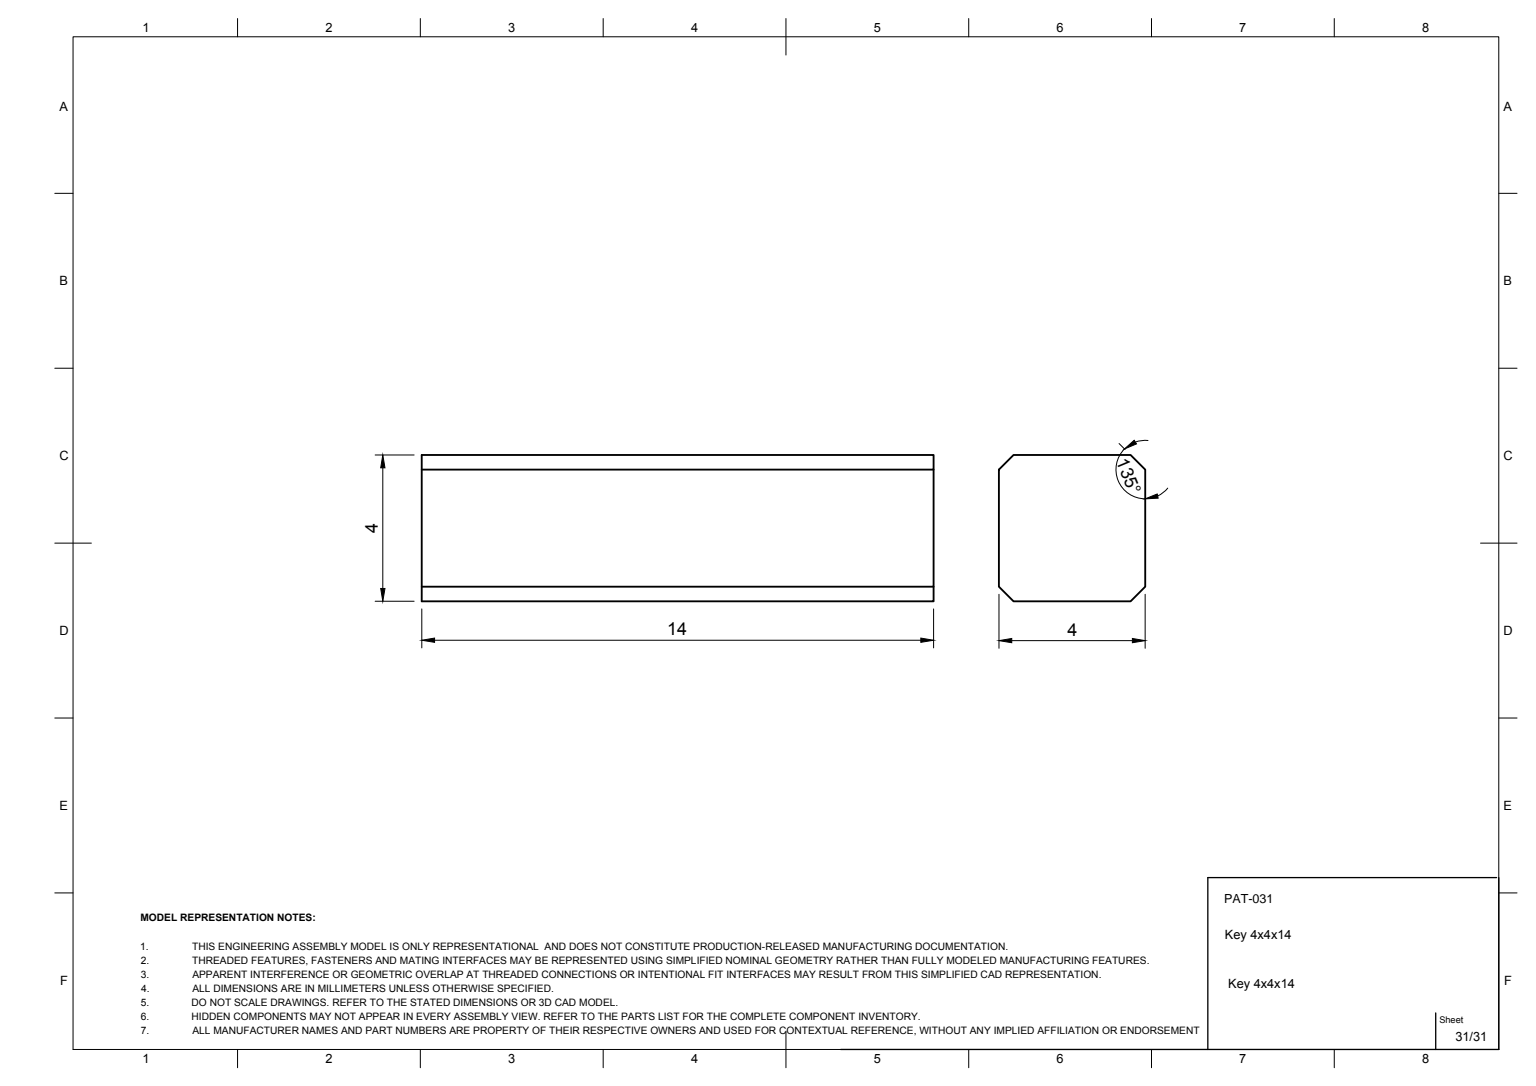
ISO-10303-21;
HEADER;
/* Generated by software containing ST-Developer
 * from STEP Tools, Inc. (www.steptools.com) 
 */

FILE_DESCRIPTION(
/* description */ ('Double-row support with tensioned shaft'),
/* implementation_level */ '2;1');

FILE_NAME(
/* name */ 'Key 4x4x14.step',
/* time_stamp */ '2026-10-27T10:50:35-07:00',
/* author */ (''),
/* organization */ (''),
/* preprocessor_version */ 'ST-DEVELOPER v20.2',
/* originating_system */ 'Autodesk Translation Framework v15.17.0.0',
/* authorisation */ '');

FILE_SCHEMA (('AUTOMOTIVE_DESIGN { 1 0 10303 214 3 1 1 }'));
ENDSEC;

DATA;
#10=MECHANICAL_DESIGN_GEOMETRIC_PRESENTATION_REPRESENTATION('',(#510),#11559);
#445=SHAPE_REPRESENTATION_RELATIONSHIP('SRR','None',#11755,#477);
#477=ADVANCED_BREP_SHAPE_REPRESENTATION('',(#540),#11557);
#510=STYLED_ITEM('',(#11967),#540);
#540=MANIFOLD_SOLID_BREP('Body1',#6358);
#898=PLANE('',#7334);
#899=PLANE('',#7335);
#900=PLANE('',#7336);
#901=PLANE('',#7337);
#902=PLANE('',#7338);
#903=PLANE('',#7339);
#904=PLANE('',#7340);
#905=PLANE('',#7341);
#906=PLANE('',#7342);
#907=PLANE('',#7343);
#1239=FACE_OUTER_BOUND('',#1719,.T.);
#1240=FACE_OUTER_BOUND('',#1720,.T.);
#1241=FACE_OUTER_BOUND('',#1721,.T.);
#1242=FACE_OUTER_BOUND('',#1722,.T.);
#1243=FACE_OUTER_BOUND('',#1723,.T.);
#1244=FACE_OUTER_BOUND('',#1724,.T.);
#1245=FACE_OUTER_BOUND('',#1725,.T.);
#1246=FACE_OUTER_BOUND('',#1726,.T.);
#1247=FACE_OUTER_BOUND('',#1727,.T.);
#1248=FACE_OUTER_BOUND('',#1728,.T.);
#1719=EDGE_LOOP('',(#5792,#5793,#5794,#5795,#5796,#5797,#5798,#5799));
#1720=EDGE_LOOP('',(#5800,#5801,#5802,#5803));
#1721=EDGE_LOOP('',(#5804,#5805,#5806,#5807));
#1722=EDGE_LOOP('',(#5808,#5809,#5810,#5811));
#1723=EDGE_LOOP('',(#5812,#5813,#5814,#5815));
#1724=EDGE_LOOP('',(#5816,#5817,#5818,#5819,#5820,#5821,#5822,#5823));
#1725=EDGE_LOOP('',(#5824,#5825,#5826,#5827));
#1726=EDGE_LOOP('',(#5828,#5829,#5830,#5831));
#1727=EDGE_LOOP('',(#5832,#5833,#5834,#5835));
#1728=EDGE_LOOP('',(#5836,#5837,#5838,#5839));
#2244=LINE('',#11375,#2791);
#2245=LINE('',#11377,#2792);
#2246=LINE('',#11379,#2793);
#2247=LINE('',#11381,#2794);
#2248=LINE('',#11383,#2795);
#2249=LINE('',#11385,#2796);
#2250=LINE('',#11387,#2797);
#2251=LINE('',#11388,#2798);
#2252=LINE('',#11391,#2799);
#2253=LINE('',#11393,#2800);
#2254=LINE('',#11394,#2801);
#2255=LINE('',#11397,#2802);
#2256=LINE('',#11398,#2803);
#2257=LINE('',#11401,#2804);
#2258=LINE('',#11402,#2805);
#2259=LINE('',#11405,#2806);
#2260=LINE('',#11406,#2807);
#2261=LINE('',#11409,#2808);
#2262=LINE('',#11411,#2809);
#2263=LINE('',#11413,#2810);
#2264=LINE('',#11414,#2811);
#2265=LINE('',#11416,#2812);
#2266=LINE('',#11418,#2813);
#2267=LINE('',#11420,#2814);
#2791=VECTOR('',#9117,1.);
#2792=VECTOR('',#9118,1.);
#2793=VECTOR('',#9119,1.);
#2794=VECTOR('',#9120,1.);
#2795=VECTOR('',#9121,1.);
#2796=VECTOR('',#9122,1.);
#2797=VECTOR('',#9123,1.);
#2798=VECTOR('',#9124,1.);
#2799=VECTOR('',#9127,1.);
#2800=VECTOR('',#9128,1.);
#2801=VECTOR('',#9129,1.);
#2802=VECTOR('',#9132,1.);
#2803=VECTOR('',#9133,1.);
#2804=VECTOR('',#9136,1.);
#2805=VECTOR('',#9137,1.);
#2806=VECTOR('',#9140,1.);
#2807=VECTOR('',#9141,1.);
#2808=VECTOR('',#9144,1.);
#2809=VECTOR('',#9145,1.);
#2810=VECTOR('',#9146,1.);
#2811=VECTOR('',#9147,1.);
#2812=VECTOR('',#9150,1.);
#2813=VECTOR('',#9153,1.);
#2814=VECTOR('',#9156,1.);
#3518=VERTEX_POINT('',#11373);
#3519=VERTEX_POINT('',#11374);
#3520=VERTEX_POINT('',#11376);
#3521=VERTEX_POINT('',#11378);
#3522=VERTEX_POINT('',#11380);
#3523=VERTEX_POINT('',#11382);
#3524=VERTEX_POINT('',#11384);
#3525=VERTEX_POINT('',#11386);
#3526=VERTEX_POINT('',#11390);
#3527=VERTEX_POINT('',#11392);
#3528=VERTEX_POINT('',#11396);
#3529=VERTEX_POINT('',#11400);
#3530=VERTEX_POINT('',#11404);
#3531=VERTEX_POINT('',#11408);
#3532=VERTEX_POINT('',#11410);
#3533=VERTEX_POINT('',#11412);
#4281=EDGE_CURVE('',#3518,#3519,#2244,.T.);
#4282=EDGE_CURVE('',#3520,#3518,#2245,.T.);
#4283=EDGE_CURVE('',#3521,#3520,#2246,.T.);
#4284=EDGE_CURVE('',#3522,#3521,#2247,.T.);
#4285=EDGE_CURVE('',#3523,#3522,#2248,.T.);
#4286=EDGE_CURVE('',#3524,#3523,#2249,.T.);
#4287=EDGE_CURVE('',#3525,#3524,#2250,.T.);
#4288=EDGE_CURVE('',#3519,#3525,#2251,.T.);
#4289=EDGE_CURVE('',#3522,#3526,#2252,.T.);
#4290=EDGE_CURVE('',#3526,#3527,#2253,.T.);
#4291=EDGE_CURVE('',#3527,#3523,#2254,.T.);
#4292=EDGE_CURVE('',#3528,#3521,#2255,.T.);
#4293=EDGE_CURVE('',#3528,#3526,#2256,.T.);
#4294=EDGE_CURVE('',#3520,#3529,#2257,.T.);
#4295=EDGE_CURVE('',#3529,#3528,#2258,.T.);
#4296=EDGE_CURVE('',#3530,#3518,#2259,.T.);
#4297=EDGE_CURVE('',#3530,#3529,#2260,.T.);
#4298=EDGE_CURVE('',#3531,#3530,#2261,.T.);
#4299=EDGE_CURVE('',#3532,#3531,#2262,.T.);
#4300=EDGE_CURVE('',#3533,#3532,#2263,.T.);
#4301=EDGE_CURVE('',#3527,#3533,#2264,.T.);
#4302=EDGE_CURVE('',#3519,#3531,#2265,.T.);
#4303=EDGE_CURVE('',#3532,#3525,#2266,.T.);
#4304=EDGE_CURVE('',#3524,#3533,#2267,.T.);
#5792=ORIENTED_EDGE('',*,*,#4281,.F.);
#5793=ORIENTED_EDGE('',*,*,#4282,.F.);
#5794=ORIENTED_EDGE('',*,*,#4283,.F.);
#5795=ORIENTED_EDGE('',*,*,#4284,.F.);
#5796=ORIENTED_EDGE('',*,*,#4285,.F.);
#5797=ORIENTED_EDGE('',*,*,#4286,.F.);
#5798=ORIENTED_EDGE('',*,*,#4287,.F.);
#5799=ORIENTED_EDGE('',*,*,#4288,.F.);
#5800=ORIENTED_EDGE('',*,*,#4285,.T.);
#5801=ORIENTED_EDGE('',*,*,#4289,.T.);
#5802=ORIENTED_EDGE('',*,*,#4290,.T.);
#5803=ORIENTED_EDGE('',*,*,#4291,.T.);
#5804=ORIENTED_EDGE('',*,*,#4284,.T.);
#5805=ORIENTED_EDGE('',*,*,#4292,.F.);
#5806=ORIENTED_EDGE('',*,*,#4293,.T.);
#5807=ORIENTED_EDGE('',*,*,#4289,.F.);
#5808=ORIENTED_EDGE('',*,*,#4283,.T.);
#5809=ORIENTED_EDGE('',*,*,#4294,.T.);
#5810=ORIENTED_EDGE('',*,*,#4295,.T.);
#5811=ORIENTED_EDGE('',*,*,#4292,.T.);
#5812=ORIENTED_EDGE('',*,*,#4282,.T.);
#5813=ORIENTED_EDGE('',*,*,#4296,.F.);
#5814=ORIENTED_EDGE('',*,*,#4297,.T.);
#5815=ORIENTED_EDGE('',*,*,#4294,.F.);
#5816=ORIENTED_EDGE('',*,*,#4290,.F.);
#5817=ORIENTED_EDGE('',*,*,#4293,.F.);
#5818=ORIENTED_EDGE('',*,*,#4295,.F.);
#5819=ORIENTED_EDGE('',*,*,#4297,.F.);
#5820=ORIENTED_EDGE('',*,*,#4298,.F.);
#5821=ORIENTED_EDGE('',*,*,#4299,.F.);
#5822=ORIENTED_EDGE('',*,*,#4300,.F.);
#5823=ORIENTED_EDGE('',*,*,#4301,.F.);
#5824=ORIENTED_EDGE('',*,*,#4281,.T.);
#5825=ORIENTED_EDGE('',*,*,#4302,.T.);
#5826=ORIENTED_EDGE('',*,*,#4298,.T.);
#5827=ORIENTED_EDGE('',*,*,#4296,.T.);
#5828=ORIENTED_EDGE('',*,*,#4288,.T.);
#5829=ORIENTED_EDGE('',*,*,#4303,.F.);
#5830=ORIENTED_EDGE('',*,*,#4299,.T.);
#5831=ORIENTED_EDGE('',*,*,#4302,.F.);
#5832=ORIENTED_EDGE('',*,*,#4287,.T.);
#5833=ORIENTED_EDGE('',*,*,#4304,.T.);
#5834=ORIENTED_EDGE('',*,*,#4300,.T.);
#5835=ORIENTED_EDGE('',*,*,#4303,.T.);
#5836=ORIENTED_EDGE('',*,*,#4286,.T.);
#5837=ORIENTED_EDGE('',*,*,#4291,.F.);
#5838=ORIENTED_EDGE('',*,*,#4301,.T.);
#5839=ORIENTED_EDGE('',*,*,#4304,.F.);
#6302=ADVANCED_FACE('',(#1239),#898,.T.);
#6303=ADVANCED_FACE('',(#1240),#899,.T.);
#6304=ADVANCED_FACE('',(#1241),#900,.T.);
#6305=ADVANCED_FACE('',(#1242),#901,.T.);
#6306=ADVANCED_FACE('',(#1243),#902,.T.);
#6307=ADVANCED_FACE('',(#1244),#903,.F.);
#6308=ADVANCED_FACE('',(#1245),#904,.T.);
#6309=ADVANCED_FACE('',(#1246),#905,.T.);
#6310=ADVANCED_FACE('',(#1247),#906,.T.);
#6311=ADVANCED_FACE('',(#1248),#907,.F.);
#6358=CLOSED_SHELL('',(#6302,#6303,#6304,#6305,#6306,#6307,#6308,#6309,
#6310,#6311));
#7333=AXIS2_PLACEMENT_3D('',#11371,#9113,#9114);
#7334=AXIS2_PLACEMENT_3D('',#11372,#9115,#9116);
#7335=AXIS2_PLACEMENT_3D('',#11389,#9125,#9126);
#7336=AXIS2_PLACEMENT_3D('',#11395,#9130,#9131);
#7337=AXIS2_PLACEMENT_3D('',#11399,#9134,#9135);
#7338=AXIS2_PLACEMENT_3D('',#11403,#9138,#9139);
#7339=AXIS2_PLACEMENT_3D('',#11407,#9142,#9143);
#7340=AXIS2_PLACEMENT_3D('',#11415,#9148,#9149);
#7341=AXIS2_PLACEMENT_3D('',#11417,#9151,#9152);
#7342=AXIS2_PLACEMENT_3D('',#11419,#9154,#9155);
#7343=AXIS2_PLACEMENT_3D('',#11421,#9157,#9158);
#9113=DIRECTION('axis',(0.,0.,1.));
#9114=DIRECTION('refdir',(1.,0.,0.));
#9115=DIRECTION('center_axis',(1.,0.,0.));
#9116=DIRECTION('ref_axis',(0.,0.,-1.));
#9117=DIRECTION('',(0.,0.707106781186547,-0.707106781186548));
#9118=DIRECTION('',(0.,1.,0.));
#9119=DIRECTION('',(0.,0.707106781186547,0.707106781186548));
#9120=DIRECTION('',(0.,0.,1.));
#9121=DIRECTION('',(0.,-0.707106781186548,0.707106781186548));
#9122=DIRECTION('',(0.,-1.,0.));
#9123=DIRECTION('',(0.,-0.707106781186548,-0.707106781186548));
#9124=DIRECTION('',(0.,0.,-1.));
#9125=DIRECTION('center_axis',(0.,-0.707106781186548,-0.707106781186548));
#9126=DIRECTION('ref_axis',(-1.,0.,0.));
#9127=DIRECTION('',(-1.,0.,0.));
#9128=DIRECTION('',(0.,0.707106781186548,-0.707106781186548));
#9129=DIRECTION('',(1.,0.,0.));
#9130=DIRECTION('center_axis',(0.,-1.,0.));
#9131=DIRECTION('ref_axis',(1.,0.,0.));
#9132=DIRECTION('',(1.,0.,0.));
#9133=DIRECTION('',(0.,0.,-1.));
#9134=DIRECTION('center_axis',(0.,-0.707106781186548,0.707106781186547));
#9135=DIRECTION('ref_axis',(1.,0.,0.));
#9136=DIRECTION('',(-1.,0.,0.));
#9137=DIRECTION('',(0.,-0.707106781186547,-0.707106781186548));
#9138=DIRECTION('center_axis',(0.,0.,1.));
#9139=DIRECTION('ref_axis',(1.,0.,0.));
#9140=DIRECTION('',(1.,0.,0.));
#9141=DIRECTION('',(0.,-1.,0.));
#9142=DIRECTION('center_axis',(1.,0.,0.));
#9143=DIRECTION('ref_axis',(0.,0.,-1.));
#9144=DIRECTION('',(0.,-0.707106781186547,0.707106781186548));
#9145=DIRECTION('',(0.,0.,1.));
#9146=DIRECTION('',(0.,0.707106781186548,0.707106781186548));
#9147=DIRECTION('',(0.,1.,0.));
#9148=DIRECTION('center_axis',(0.,0.707106781186548,0.707106781186547));
#9149=DIRECTION('ref_axis',(1.,0.,0.));
#9150=DIRECTION('',(-1.,0.,0.));
#9151=DIRECTION('center_axis',(0.,1.,0.));
#9152=DIRECTION('ref_axis',(-1.,0.,0.));
#9153=DIRECTION('',(1.,0.,0.));
#9154=DIRECTION('center_axis',(0.,0.707106781186548,-0.707106781186548));
#9155=DIRECTION('ref_axis',(-1.,0.,0.));
#9156=DIRECTION('',(-1.,0.,0.));
#9157=DIRECTION('center_axis',(0.,0.,1.));
#9158=DIRECTION('ref_axis',(1.,0.,0.));
#11371=CARTESIAN_POINT('',(0.,0.,0.));
#11372=CARTESIAN_POINT('Origin',(0.7,0.,0.25));
#11373=CARTESIAN_POINT('',(0.7,0.16,0.4));
#11374=CARTESIAN_POINT('',(0.7,0.2,0.36));
#11375=CARTESIAN_POINT('',(0.7,0.1675,0.3925));
#11376=CARTESIAN_POINT('',(0.7,-0.16,0.4));
#11377=CARTESIAN_POINT('',(0.7,0.,0.4));
#11378=CARTESIAN_POINT('',(0.7,-0.2,0.36));
#11379=CARTESIAN_POINT('',(0.7,-0.1675,0.3925));
#11380=CARTESIAN_POINT('',(0.7,-0.2,0.04));
#11381=CARTESIAN_POINT('',(0.7,-0.2,0.125));
#11382=CARTESIAN_POINT('',(0.7,-0.16,0.));
#11383=CARTESIAN_POINT('',(0.7,-0.1925,0.0325));
#11384=CARTESIAN_POINT('',(0.7,0.16,0.));
#11385=CARTESIAN_POINT('',(0.7,0.,0.));
#11386=CARTESIAN_POINT('',(0.7,0.2,0.04));
#11387=CARTESIAN_POINT('',(0.7,0.1925,0.0325));
#11388=CARTESIAN_POINT('',(0.7,0.2,0.125));
#11389=CARTESIAN_POINT('Origin',(-0.4,-0.18,0.02));
#11390=CARTESIAN_POINT('',(-0.7,-0.2,0.04));
#11391=CARTESIAN_POINT('',(-0.4,-0.2,0.04));
#11392=CARTESIAN_POINT('',(-0.7,-0.16,0.));
#11393=CARTESIAN_POINT('',(-0.7,-0.1925,0.0325));
#11394=CARTESIAN_POINT('',(-0.4,-0.16,0.));
#11395=CARTESIAN_POINT('Origin',(-0.8,-0.2,0.));
#11396=CARTESIAN_POINT('',(-0.7,-0.2,0.36));
#11397=CARTESIAN_POINT('',(-0.4,-0.2,0.36));
#11398=CARTESIAN_POINT('',(-0.7,-0.2,0.125));
#11399=CARTESIAN_POINT('Origin',(-0.4,-0.18,0.38));
#11400=CARTESIAN_POINT('',(-0.7,-0.16,0.4));
#11401=CARTESIAN_POINT('',(-0.4,-0.16,0.4));
#11402=CARTESIAN_POINT('',(-0.7,-0.1675,0.3925));
#11403=CARTESIAN_POINT('Origin',(0.,0.,0.4));
#11404=CARTESIAN_POINT('',(-0.7,0.16,0.4));
#11405=CARTESIAN_POINT('',(0.4,0.16,0.4));
#11406=CARTESIAN_POINT('',(-0.7,0.,0.4));
#11407=CARTESIAN_POINT('Origin',(-0.7,0.,0.25));
#11408=CARTESIAN_POINT('',(-0.7,0.2,0.36));
#11409=CARTESIAN_POINT('',(-0.7,0.1675,0.3925));
#11410=CARTESIAN_POINT('',(-0.7,0.2,0.04));
#11411=CARTESIAN_POINT('',(-0.7,0.2,0.125));
#11412=CARTESIAN_POINT('',(-0.7,0.16,0.));
#11413=CARTESIAN_POINT('',(-0.7,0.1925,0.0325));
#11414=CARTESIAN_POINT('',(-0.7,0.,0.));
#11415=CARTESIAN_POINT('Origin',(0.4,0.18,0.38));
#11416=CARTESIAN_POINT('',(0.4,0.2,0.36));
#11417=CARTESIAN_POINT('Origin',(0.8,0.2,0.));
#11418=CARTESIAN_POINT('',(0.4,0.2,0.04));
#11419=CARTESIAN_POINT('Origin',(0.4,0.18,0.02));
#11420=CARTESIAN_POINT('',(0.4,0.16,0.));
#11421=CARTESIAN_POINT('Origin',(0.,0.,0.));
#11520=UNCERTAINTY_MEASURE_WITH_UNIT(LENGTH_MEASURE(0.001),#11560,
'DISTANCE_ACCURACY_VALUE',
'Maximum model space distance between geometric entities at asserted c
onnectivities');
#11522=UNCERTAINTY_MEASURE_WITH_UNIT(LENGTH_MEASURE(0.001),#11560,
'DISTANCE_ACCURACY_VALUE',
'Maximum model space distance between geometric entities at asserted c
onnectivities');
#11557=(
GEOMETRIC_REPRESENTATION_CONTEXT(3)
GLOBAL_UNCERTAINTY_ASSIGNED_CONTEXT((#11520))
GLOBAL_UNIT_ASSIGNED_CONTEXT((#11560,#11562,#11563))
REPRESENTATION_CONTEXT('','3D')
);
#11559=(
GEOMETRIC_REPRESENTATION_CONTEXT(3)
GLOBAL_UNCERTAINTY_ASSIGNED_CONTEXT((#11522))
GLOBAL_UNIT_ASSIGNED_CONTEXT((#11560,#11562,#11563))
REPRESENTATION_CONTEXT('','3D')
);
#11560=(
LENGTH_UNIT()
NAMED_UNIT(*)
SI_UNIT(.CENTI.,.METRE.)
);
#11562=(
NAMED_UNIT(*)
PLANE_ANGLE_UNIT()
SI_UNIT($,.RADIAN.)
);
#11563=(
NAMED_UNIT(*)
SI_UNIT($,.STERADIAN.)
SOLID_ANGLE_UNIT()
);
#11598=SHAPE_DEFINITION_REPRESENTATION(#11709,#11755);
#11709=PRODUCT_DEFINITION_SHAPE('',$,#11792);
#11755=SHAPE_REPRESENTATION('',(#7333),#11557);
#11757=PRODUCT_DEFINITION_CONTEXT('part definition',#11867,'design');
#11792=PRODUCT_DEFINITION('Key 4x4x14','Key 4x4x14',#11828,#11757);
#11828=PRODUCT_DEFINITION_FORMATION('',$,#11903);
#11867=APPLICATION_CONTEXT(
'Core Data for Automotive Mechanical Design Process');
#11868=PRODUCT_CONTEXT('part definition',#11867,'mechanical');
#11903=PRODUCT('Key 4x4x14','Key 4x4x14','Key 4x4x14',(#11868));
#11961=COLOUR_RGB('Grey',0.48,0.52,0.57);
#11962=FILL_AREA_STYLE_COLOUR('',#11961);
#11963=FILL_AREA_STYLE('',(#11962));
#11964=SURFACE_STYLE_FILL_AREA(#11963);
#11965=SURFACE_SIDE_STYLE('',(#11964));
#11966=SURFACE_STYLE_USAGE(.BOTH.,#11965);
#11967=PRESENTATION_STYLE_ASSIGNMENT((#11966));
ENDSEC;
END-ISO-10303-21;
